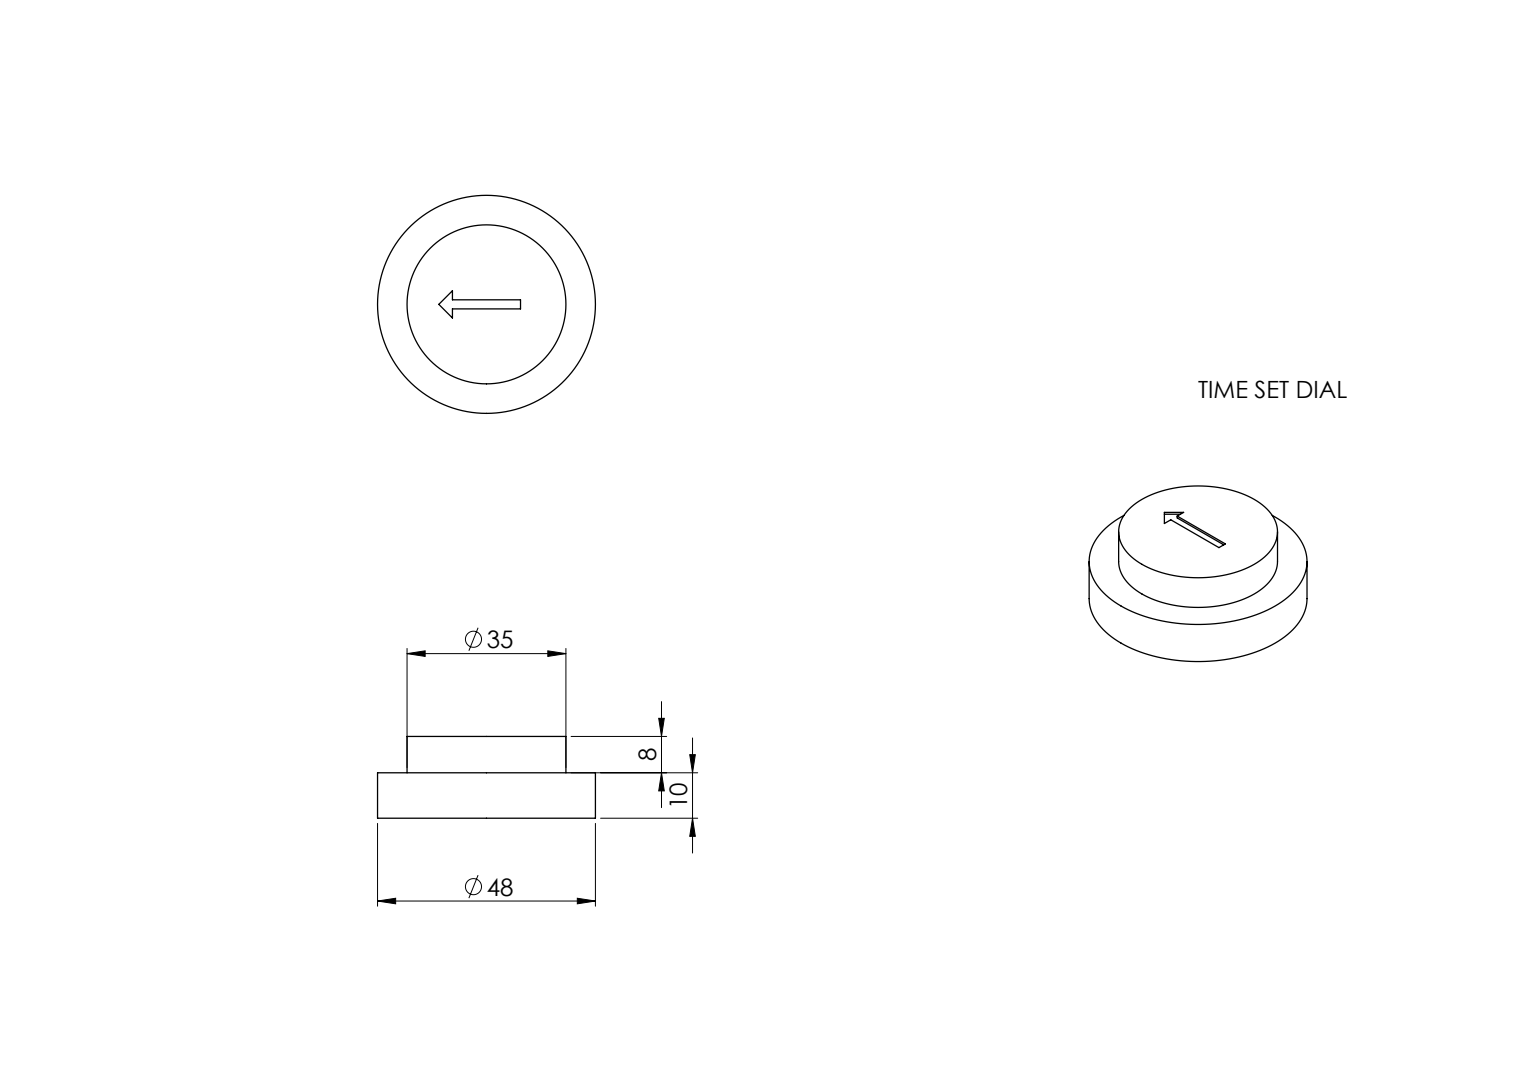
ISO-10303-21;
HEADER;
FILE_DESCRIPTION (('STEP AP214'),
    '1' );
FILE_NAME ('time set dial.step',
    '2026-10-24T15:06:47',
    ( '' ),
    ( '' ),
    'SwSTEP 2.0',
    'SolidWorks 2026',
    '' );
FILE_SCHEMA (( 'AUTOMOTIVE_DESIGN' ));
ENDSEC;

DATA;
#24=FACE_OUTER_BOUND ( 'NONE', #4526, .T. ) ;
#82=AXIS2_PLACEMENT_3D ( 'NONE', #9543, #4773, #8119 ) ;
#92=ORIENTED_EDGE ( 'NONE', *, *, #2350, .T. ) ;
#107=DIRECTION ( 'NONE',  ( 0.000000000000000000, 0.000000000000000000, 1.000000000000000000 ) ) ;
#109=DIRECTION ( 'NONE',  ( 4.336808689942017736E-16, 0.000000000000000000, -1.000000000000000000 ) ) ;
#117=FACE_OUTER_BOUND ( 'NONE', #7334, .T. ) ;
#145=LINE ( 'NONE', #6521, #2502 ) ;
#146=DIRECTION ( 'NONE',  ( -1.000000000000000000, -0.000000000000000000, -0.000000000000000000 ) ) ;
#204=VECTOR ( 'NONE', #9185, 1000.000000000000000 ) ;
#241=ORIENTED_EDGE ( 'NONE', *, *, #4209, .F. ) ;
#262=LINE ( 'NONE', #2027, #6876 ) ;
#291=DIRECTION ( 'NONE',  ( -0.000000000000000000, 1.000000000000000000, -0.000000000000000000 ) ) ;
#295=CIRCLE ( 'NONE', #9511, 17.50000000000000355 ) ;
#305=AXIS2_PLACEMENT_3D ( 'NONE', #9568, #7104, #7052 ) ;
#342=CARTESIAN_POINT ( 'NONE',  ( -10.49999999999999822, 105.0000000000000142, 0.000000000000000000 ) ) ;
#376=CARTESIAN_POINT ( 'NONE',  ( -7.500000000000000000, 105.0000000000000142, 1.000000000000000222 ) ) ;
#379=AXIS2_PLACEMENT_3D ( 'NONE', #1311, #2259, #3050 ) ;
#382=ORIENTED_EDGE ( 'NONE', *, *, #7990, .T. ) ;
#469=LINE ( 'NONE', #7744, #6933 ) ;
#510=STYLED_ITEM('',(#10415),#6220);
#513=PLANE ( 'NONE',  #9858 ) ;
#568=CARTESIAN_POINT ( 'NONE',  ( 7.500000000000000000, 104.5000000000000142, -0.9999999999999997780 ) ) ;
#570=VERTEX_POINT ( 'NONE', #7174 ) ;
#582=PLANE ( 'NONE',  #8912 ) ;
#591=LINE ( 'NONE', #8435, #9453 ) ;
#592=EDGE_CURVE ( 'NONE', #4647, #7571, #9632, .T. ) ;
#595=ORIENTED_EDGE ( 'NONE', *, *, #7990, .F. ) ;
#619=ORIENTED_EDGE ( 'NONE', *, *, #3800, .T. ) ;
#638=ADVANCED_FACE ( 'NONE', ( #8160 ), #1037, .F. ) ;
#674=ORIENTED_EDGE ( 'NONE', *, *, #7210, .F. ) ;
#677=EDGE_LOOP ( 'NONE', ( #674, #3279, #3413, #7812 ) ) ;
#714=ORIENTED_EDGE ( 'NONE', *, *, #1547, .T. ) ;
#726=PLANE ( 'NONE',  #305 ) ;
#741=DIRECTION ( 'NONE',  ( -0.7071067811865476838, 0.000000000000000000, -0.7071067811865474617 ) ) ;
#765=CARTESIAN_POINT ( 'NONE',  ( -7.500000000000000000, 104.5000000000000142, -3.000000000000000000 ) ) ;
#771=VECTOR ( 'NONE', #1661, 1000.000000000000000 ) ;
#781=DIRECTION ( 'NONE',  ( 0.000000000000000000, 1.000000000000000000, 0.000000000000000000 ) ) ;
#794=LINE ( 'NONE', #1520, #8161 ) ;
#808=ORIENTED_EDGE ( 'NONE', *, *, #8492, .T. ) ;
#814=AXIS2_PLACEMENT_3D ( 'NONE', #8760, #6354, #2424 ) ;
#816=DIRECTION ( 'NONE',  ( 0.000000000000000000, 1.000000000000000000, 0.000000000000000000 ) ) ;
#857=ORIENTED_EDGE ( 'NONE', *, *, #9277, .F. ) ;
#864=LINE ( 'NONE', #8915, #7733 ) ;
#906=VERTEX_POINT ( 'NONE', #10349 ) ;
#944=ADVANCED_FACE ( 'NONE', ( #24 ), #4011, .F. ) ;
#960=DIRECTION ( 'NONE',  ( -0.000000000000000000, -1.000000000000000000, -0.000000000000000000 ) ) ;
#1026=PLANE ( 'NONE',  #6043 ) ;
#1036=AXIS2_PLACEMENT_3D ( 'NONE', #6464, #816, #8134 ) ;
#1037=PLANE ( 'NONE',  #7108 ) ;
#1061=VERTEX_POINT ( 'NONE', #376 ) ;
#1093=AXIS2_PLACEMENT_3D ( 'NONE', #5684, #7295, #9604 ) ;
#1097=DIRECTION ( 'NONE',  ( -0.000000000000000000, -1.000000000000000000, -0.000000000000000000 ) ) ;
#1119=LINE ( 'NONE', #1995, #2870 ) ;
#1179=DIRECTION ( 'NONE',  ( 0.7071067811865473507, 0.000000000000000000, 0.7071067811865477948 ) ) ;
#1211=SHAPE_REPRESENTATION_RELATIONSHIP ( 'NONE' , 'NONE' ,  #5481, #6379 ) ;
#1262=CARTESIAN_POINT ( 'NONE',  ( 0.000000000000000000, 97.00000000000000000, 0.000000000000000000 ) ) ;
#1292=CARTESIAN_POINT ( 'NONE',  ( 0.000000000000000000, 105.0000000000000142, 0.000000000000000000 ) ) ;
#1297=ORIENTED_EDGE ( 'NONE', *, *, #1332, .F. ) ;
#1308=UNCERTAINTY_MEASURE_WITH_UNIT (LENGTH_MEASURE( 1.000000000000000082E-05 ), #6022, 'distance_accuracy_value', 'NONE');
#1311=CARTESIAN_POINT ( 'NONE',  ( 0.000000000000000000, 105.0000000000000142, 0.000000000000000000 ) ) ;
#1332=EDGE_CURVE ( 'NONE', #9169, #7011, #4267, .T. ) ;
#1333=PRODUCT ( 'time set dial', 'time set dial', '', ( #2137 ) ) ;
#1352=EDGE_CURVE ( 'NONE', #1061, #570, #8955, .T. ) ;
#1361=CARTESIAN_POINT ( 'NONE',  ( 2.939152317953648289E-15, 97.00000000000000000, 24.00000000000000355 ) ) ;
#1376=ORIENTED_EDGE ( 'NONE', *, *, #1332, .T. ) ;
#1396=( GEOMETRIC_REPRESENTATION_CONTEXT ( 3 ) GLOBAL_UNCERTAINTY_ASSIGNED_CONTEXT ( ( #3296 ) ) GLOBAL_UNIT_ASSIGNED_CONTEXT ( ( #7429, #6752, #9893 ) ) REPRESENTATION_CONTEXT ( 'NONE', 'WORKASPACE' ) );
#1397=PLANE ( 'NONE',  #7889 ) ;
#1403=FACE_OUTER_BOUND ( 'NONE', #9984, .T. ) ;
#1500=CARTESIAN_POINT ( 'NONE',  ( 0.000000000000000000, 105.0000000000000142, -17.50000000000000355 ) ) ;
#1520=CARTESIAN_POINT ( 'NONE',  ( 7.500000000000000000, 104.5000000000000142, 1.000000000000000222 ) ) ;
#1536=ORIENTED_EDGE ( 'NONE', *, *, #7153, .T. ) ;
#1545=ORIENTED_EDGE ( 'NONE', *, *, #9344, .F. ) ;
#1547=EDGE_CURVE ( 'NONE', #7571, #1061, #262, .T. ) ;
#1622=ORIENTED_EDGE ( 'NONE', *, *, #7157, .F. ) ;
#1661=DIRECTION ( 'NONE',  ( -0.000000000000000000, 1.000000000000000000, -0.000000000000000000 ) ) ;
#1675=DIRECTION ( 'NONE',  ( 0.000000000000000000, 0.000000000000000000, -1.000000000000000000 ) ) ;
#1681=DIRECTION ( 'NONE',  ( 0.000000000000000000, 1.000000000000000000, 0.000000000000000000 ) ) ;
#1704=AXIS2_PLACEMENT_3D ( 'NONE', #8807, #9734, #5767 ) ;
#1709=DIRECTION ( 'NONE',  ( 0.000000000000000000, -0.000000000000000000, 1.000000000000000000 ) ) ;
#1720=AXIS2_PLACEMENT_3D ( 'NONE', #9929, #1813, #4230 ) ;
#1727=ORIENTED_EDGE ( 'NONE', *, *, #7157, .T. ) ;
#1743=ORIENTED_EDGE ( 'NONE', *, *, #8141, .F. ) ;
#1753=CARTESIAN_POINT ( 'NONE',  ( -7.500000000000000000, 104.5000000000000142, -3.000000000000000000 ) ) ;
#1761=LINE ( 'NONE', #9094, #8320 ) ;
#1767=CIRCLE ( 'NONE', #1936, 24.00000000000000355 ) ;
#1772=CARTESIAN_POINT ( 'NONE',  ( -7.500000000000000000, 105.0000000000000142, 1.000000000000000222 ) ) ;
#1813=DIRECTION ( 'NONE',  ( 0.000000000000000000, -1.000000000000000000, 0.000000000000000000 ) ) ;
#1837=ORIENTED_EDGE ( 'NONE', *, *, #10080, .F. ) ;
#1865=ORIENTED_EDGE ( 'NONE', *, *, #1352, .T. ) ;
#1898=LINE ( 'NONE', #1753, #5297 ) ;
#1904=DIRECTION ( 'NONE',  ( -0.7071067811865477948, 0.000000000000000000, 0.7071067811865473507 ) ) ;
#1936=AXIS2_PLACEMENT_3D ( 'NONE', #4316, #1681, #9133 ) ;
#1963=( NAMED_UNIT ( * ) PLANE_ANGLE_UNIT ( ) SI_UNIT ( $, .RADIAN. ) );
#1995=CARTESIAN_POINT ( 'NONE',  ( -7.500000000000000000, 104.5000000000000142, -0.9999999999999997780 ) ) ;
#2021=EDGE_CURVE ( 'NONE', #3170, #3531, #7292, .T. ) ;
#2027=CARTESIAN_POINT ( 'NONE',  ( -7.500000000000000000, 104.5000000000000142, 1.000000000000000222 ) ) ;
#2042=PRESENTATION_STYLE_ASSIGNMENT (( #5414 ) ) ;
#2090=AXIS2_PLACEMENT_3D ( 'NONE', #7524, #1097, #5813 ) ;
#2117=AXIS2_PLACEMENT_3D ( 'NONE', #2132, #2192, #6052 ) ;
#2131=VERTEX_POINT ( 'NONE', #2333 ) ;
#2132=CARTESIAN_POINT ( 'NONE',  ( 0.000000000000000000, 87.00000000000001421, 0.000000000000000000 ) ) ;
#2137=PRODUCT_CONTEXT ( 'NONE', #5679, 'mechanical' ) ;
#2149=CARTESIAN_POINT ( 'NONE',  ( -10.49999999999999822, 104.5000000000000142, 0.000000000000000000 ) ) ;
#2158=EDGE_CURVE ( 'NONE', #3256, #2131, #3898, .T. ) ;
#2192=DIRECTION ( 'NONE',  ( 0.000000000000000000, 1.000000000000000000, 0.000000000000000000 ) ) ;
#2259=DIRECTION ( 'NONE',  ( 0.000000000000000000, 1.000000000000000000, 0.000000000000000000 ) ) ;
#2275=ORIENTED_EDGE ( 'NONE', *, *, #6709, .F. ) ;
#2290=CARTESIAN_POINT ( 'NONE',  ( -10.49999999999999822, 104.5000000000000142, 0.000000000000000000 ) ) ;
#2333=CARTESIAN_POINT ( 'NONE',  ( 2.143131898507868643E-15, 97.00000000000000000, 17.50000000000000355 ) ) ;
#2350=EDGE_CURVE ( 'NONE', #6922, #2378, #7401, .T. ) ;
#2360=ADVANCED_FACE ( 'NONE', ( #9865 ), #1026, .F. ) ;
#2378=VERTEX_POINT ( 'NONE', #7452 ) ;
#2393=DIRECTION ( 'NONE',  ( 0.7071067811865473507, 0.000000000000000000, 0.7071067811865477948 ) ) ;
#2394=CARTESIAN_POINT ( 'NONE',  ( 0.000000000000000000, 105.0000000000000142, -17.50000000000000355 ) ) ;
#2424=DIRECTION ( 'NONE',  ( 0.000000000000000000, 0.000000000000000000, -1.000000000000000000 ) ) ;
#2438=EDGE_LOOP ( 'NONE', ( #1622, #7880, #10051, #8233 ) ) ;
#2440=ORIENTED_EDGE ( 'NONE', *, *, #10080, .T. ) ;
#2451=( NAMED_UNIT ( * ) SI_UNIT ( $, .STERADIAN. ) SOLID_ANGLE_UNIT ( ) );
#2464=CARTESIAN_POINT ( 'NONE',  ( -10.49999999999999822, 105.0000000000000142, 0.000000000000000000 ) ) ;
#2466=CARTESIAN_POINT ( 'NONE',  ( -7.500000000000000888, 104.5000000000000142, 3.000000000000000000 ) ) ;
#2501=DIRECTION ( 'NONE',  ( -0.000000000000000000, -0.000000000000000000, -1.000000000000000000 ) ) ;
#2502=VECTOR ( 'NONE', #2501, 1000.000000000000000 ) ;
#2516=CARTESIAN_POINT ( 'NONE',  ( 7.500000000000000000, 104.5000000000000142, 1.000000000000000222 ) ) ;
#2693=EDGE_LOOP ( 'NONE', ( #5365, #6331, #9868, #9244 ) ) ;
#2699=ORIENTED_EDGE ( 'NONE', *, *, #7028, .T. ) ;
#2728=COLOUR_RGB ( '',0.8941176470588234615, 0.8941176470588234615, 0.8941176470588234615 ) ;
#2808=CARTESIAN_POINT ( 'NONE',  ( -10.49999999999999822, 104.5000000000000142, 0.000000000000000000 ) ) ;
#2851=ADVANCED_FACE ( 'NONE', ( #10321, #3724 ), #3106, .T. ) ;
#2861=ADVANCED_FACE ( 'NONE', ( #3775 ), #582, .F. ) ;
#2870=VECTOR ( 'NONE', #5879, 1000.000000000000000 ) ;
#2932=CARTESIAN_POINT ( 'NONE',  ( -7.500000000000000888, 104.5000000000000142, 3.000000000000000000 ) ) ;
#2959=ORIENTED_EDGE ( 'NONE', *, *, #2158, .F. ) ;
#2981=CARTESIAN_POINT ( 'NONE',  ( -7.500000000000000000, 104.5000000000000142, -0.9999999999999997780 ) ) ;
#2999=VECTOR ( 'NONE', #146, 1000.000000000000000 ) ;
#3009=SURFACE_SIDE_STYLE ('',( #5181 ) ) ;
#3050=DIRECTION ( 'NONE',  ( 0.000000000000000000, -0.000000000000000000, 1.000000000000000000 ) ) ;
#3055=ADVANCED_FACE ( 'NONE', ( #9193 ), #8257, .F. ) ;
#3086=ORIENTED_EDGE ( 'NONE', *, *, #3800, .F. ) ;
#3103=PRODUCT_DEFINITION_CONTEXT ( 'detailed design', #10152, 'design' ) ;
#3106=PLANE ( 'NONE',  #379 ) ;
#3143=DIRECTION ( 'NONE',  ( 0.000000000000000000, 0.000000000000000000, 1.000000000000000000 ) ) ;
#3170=VERTEX_POINT ( 'NONE', #10067 ) ;
#3183=DIRECTION ( 'NONE',  ( -0.000000000000000000, -1.000000000000000000, -0.000000000000000000 ) ) ;
#3256=VERTEX_POINT ( 'NONE', #8560 ) ;
#3279=ORIENTED_EDGE ( 'NONE', *, *, #6211, .F. ) ;
#3296=UNCERTAINTY_MEASURE_WITH_UNIT (LENGTH_MEASURE( 1.000000000000000082E-05 ), #7429, 'distance_accuracy_value', 'NONE');
#3327=DIRECTION ( 'NONE',  ( 0.000000000000000000, 0.000000000000000000, 1.000000000000000000 ) ) ;
#3329=EDGE_CURVE ( 'NONE', #9169, #9715, #864, .T. ) ;
#3398=CYLINDRICAL_SURFACE ( 'NONE', #2090, 17.50000000000000355 ) ;
#3401=ORIENTED_EDGE ( 'NONE', *, *, #592, .T. ) ;
#3413=ORIENTED_EDGE ( 'NONE', *, *, #9332, .T. ) ;
#3442=PRODUCT_DEFINITION ( 'UNKNOWN', '', #8308, #3103 ) ;
#3453=AXIS2_PLACEMENT_3D ( 'NONE', #4025, #781, #3143 ) ;
#3457=EDGE_LOOP ( 'NONE', ( #9362, #5000, #7737, #2440 ) ) ;
#3495=VERTEX_POINT ( 'NONE', #7941 ) ;
#3527=CARTESIAN_POINT ( 'NONE',  ( -10.49999999999999822, 105.0000000000000142, 0.000000000000000000 ) ) ;
#3531=VERTEX_POINT ( 'NONE', #10354 ) ;
#3541=LINE ( 'NONE', #2516, #9546 ) ;
#3580=ADVANCED_FACE ( 'NONE', ( #5380 ), #1397, .F. ) ;
#3611=DIRECTION ( 'NONE',  ( -0.000000000000000000, 1.000000000000000000, -0.000000000000000000 ) ) ;
#3618=AXIS2_PLACEMENT_3D ( 'NONE', #3964, #9514, #3327 ) ;
#3648=CIRCLE ( 'NONE', #7997, 17.50000000000000355 ) ;
#3653=DIRECTION ( 'NONE',  ( 0.000000000000000000, 0.000000000000000000, -1.000000000000000000 ) ) ;
#3680=EDGE_LOOP ( 'NONE', ( #9796, #7586, #241, #5335, #3732, #5188, #9994 ) ) ;
#3724=FACE_OUTER_BOUND ( 'NONE', #9122, .T. ) ;
#3732=ORIENTED_EDGE ( 'NONE', *, *, #7105, .F. ) ;
#3762=PLANE ( 'NONE',  #2117 ) ;
#3775=FACE_OUTER_BOUND ( 'NONE', #9335, .T. ) ;
#3781=ORIENTED_EDGE ( 'NONE', *, *, #8141, .T. ) ;
#3790=ORIENTED_EDGE ( 'NONE', *, *, #8261, .F. ) ;
#3800=EDGE_CURVE ( 'NONE', #7095, #2378, #1119, .T. ) ;
#3801=CIRCLE ( 'NONE', #3618, 24.00000000000000355 ) ;
#3813=ORIENTED_EDGE ( 'NONE', *, *, #2021, .T. ) ;
#3822=VECTOR ( 'NONE', #8896, 1000.000000000000000 ) ;
#3893=ORIENTED_EDGE ( 'NONE', *, *, #7153, .F. ) ;
#3898=CIRCLE ( 'NONE', #1036, 17.50000000000000355 ) ;
#3934=DIRECTION ( 'NONE',  ( -0.7071067811865474617, 0.000000000000000000, 0.7071067811865476838 ) ) ;
#3964=CARTESIAN_POINT ( 'NONE',  ( 0.000000000000000000, 87.00000000000001421, 0.000000000000000000 ) ) ;
#3985=DIRECTION ( 'NONE',  ( 0.000000000000000000, 1.000000000000000000, 0.000000000000000000 ) ) ;
#4011=PLANE ( 'NONE',  #1093 ) ;
#4025=CARTESIAN_POINT ( 'NONE',  ( 0.000000000000000000, 87.00000000000001421, 0.000000000000000000 ) ) ;
#4055=VECTOR ( 'NONE', #4095, 1000.000000000000000 ) ;
#4068=MECHANICAL_DESIGN_GEOMETRIC_PRESENTATION_REPRESENTATION('',(#7237),#7083);
#4095=DIRECTION ( 'NONE',  ( 1.000000000000000000, 0.000000000000000000, 0.000000000000000000 ) ) ;
#4154=DIRECTION ( 'NONE',  ( 0.000000000000000000, 0.000000000000000000, 1.000000000000000000 ) ) ;
#4169=ORIENTED_EDGE ( 'NONE', *, *, #9725, .T. ) ;
#4192=CARTESIAN_POINT ( 'NONE',  ( 0.000000000000000000, 97.00000000000000000, 0.000000000000000000 ) ) ;
#4209=EDGE_CURVE ( 'NONE', #4294, #1061, #591, .T. ) ;
#4216=FACE_OUTER_BOUND ( 'NONE', #6879, .T. ) ;
#4230=DIRECTION ( 'NONE',  ( 0.000000000000000000, -0.000000000000000000, -1.000000000000000000 ) ) ;
#4263=ADVANCED_FACE ( 'NONE', ( #117 ), #5669, .T. ) ;
#4267=CIRCLE ( 'NONE', #1704, 24.00000000000000355 ) ;
#4279=DIRECTION ( 'NONE',  ( 1.000000000000000000, 0.000000000000000000, 4.336808689942017736E-16 ) ) ;
#4294=VERTEX_POINT ( 'NONE', #9639 ) ;
#4311=AXIS2_PLACEMENT_3D ( 'NONE', #9712, #7397, #1709 ) ;
#4316=CARTESIAN_POINT ( 'NONE',  ( 0.000000000000000000, 97.00000000000000000, 0.000000000000000000 ) ) ;
#4420=CARTESIAN_POINT ( 'NONE',  ( -10.49999999999999822, 104.5000000000000142, 0.000000000000000000 ) ) ;
#4451=FACE_OUTER_BOUND ( 'NONE', #8412, .T. ) ;
#4470=CARTESIAN_POINT ( 'NONE',  ( 7.500000000000000000, 104.5000000000000142, -0.9999999999999997780 ) ) ;
#4472=CARTESIAN_POINT ( 'NONE',  ( 0.000000000000000000, 97.00000000000000000, -24.00000000000000355 ) ) ;
#4526=EDGE_LOOP ( 'NONE', ( #5095, #6153, #3790, #619 ) ) ;
#4563=( NAMED_UNIT ( * ) PLANE_ANGLE_UNIT ( ) SI_UNIT ( $, .RADIAN. ) );
#4572=VECTOR ( 'NONE', #291, 1000.000000000000000 ) ;
#4647=VERTEX_POINT ( 'NONE', #2932 ) ;
#4773=DIRECTION ( 'NONE',  ( -0.000000000000000000, -1.000000000000000000, -0.000000000000000000 ) ) ;
#4796=ORIENTED_EDGE ( 'NONE', *, *, #6012, .F. ) ;
#4797=VECTOR ( 'NONE', #109, 1000.000000000000000 ) ;
#4903=VECTOR ( 'NONE', #1179, 999.9999999999998863 ) ;
#4930=DIRECTION ( 'NONE',  ( 0.000000000000000000, 0.000000000000000000, -1.000000000000000000 ) ) ;
#4934=FILL_AREA_STYLE_COLOUR ( '', #2728 ) ;
#4961=CARTESIAN_POINT ( 'NONE',  ( -7.500000000000000888, 104.5000000000000142, 3.000000000000000000 ) ) ;
#5000=ORIENTED_EDGE ( 'NONE', *, *, #5457, .F. ) ;
#5055=AXIS2_PLACEMENT_3D ( 'NONE', #9842, #4154, #9744 ) ;
#5095=ORIENTED_EDGE ( 'NONE', *, *, #6474, .T. ) ;
#5107=EDGE_CURVE ( 'NONE', #7571, #3495, #469, .T. ) ;
#5127=LINE ( 'NONE', #6551, #7444 ) ;
#5181=SURFACE_STYLE_FILL_AREA ( #8132 ) ;
#5188=ORIENTED_EDGE ( 'NONE', *, *, #6474, .F. ) ;
#5200=EDGE_LOOP ( 'NONE', ( #1536, #9622, #9646, #7764, #808, #3401, #7707 ) ) ;
#5297=VECTOR ( 'NONE', #9030, 1000.000000000000000 ) ;
#5299=EDGE_LOOP ( 'NONE', ( #4169, #595, #3893, #9829 ) ) ;
#5330=DIRECTION ( 'NONE',  ( -1.000000000000000000, 0.000000000000000000, -0.000000000000000000 ) ) ;
#5335=ORIENTED_EDGE ( 'NONE', *, *, #10165, .F. ) ;
#5365=ORIENTED_EDGE ( 'NONE', *, *, #4209, .T. ) ;
#5380=FACE_OUTER_BOUND ( 'NONE', #5299, .T. ) ;
#5414=SURFACE_STYLE_USAGE ( .BOTH. , #3009 ) ;
#5457=EDGE_CURVE ( 'NONE', #4647, #4294, #6160, .T. ) ;
#5481=SHAPE_REPRESENTATION ( 'time set dial', ( #5055 ), #1396 ) ;
#5487=LINE ( 'NONE', #8879, #8970 ) ;
#5537=CIRCLE ( 'NONE', #8039, 17.50000000000000355 ) ;
#5621=FACE_OUTER_BOUND ( 'NONE', #2438, .T. ) ;
#5635=AXIS2_PLACEMENT_3D ( 'NONE', #1262, #9889, #7638 ) ;
#5669=CYLINDRICAL_SURFACE ( 'NONE', #82, 24.00000000000000355 ) ;
#5679=APPLICATION_CONTEXT ( 'automotive_design' ) ;
#5684=CARTESIAN_POINT ( 'NONE',  ( -7.500000000000000000, 104.5000000000000142, -3.000000000000000000 ) ) ;
#5711=ADVANCED_FACE ( 'NONE', ( #7474 ), #3398, .T. ) ;
#5767=DIRECTION ( 'NONE',  ( 0.000000000000000000, 0.000000000000000000, 1.000000000000000000 ) ) ;
#5792=VECTOR ( 'NONE', #2393, 999.9999999999998863 ) ;
#5799=DIRECTION ( 'NONE',  ( -0.000000000000000000, 1.000000000000000000, -0.000000000000000000 ) ) ;
#5813=DIRECTION ( 'NONE',  ( 0.000000000000000000, 0.000000000000000000, -1.000000000000000000 ) ) ;
#5835=CARTESIAN_POINT ( 'NONE',  ( -7.500000000000000000, 104.5000000000000142, -0.9999999999999997780 ) ) ;
#5879=DIRECTION ( 'NONE',  ( -0.000000000000000000, 1.000000000000000000, -0.000000000000000000 ) ) ;
#6011=ORIENTED_EDGE ( 'NONE', *, *, #3329, .F. ) ;
#6012=EDGE_CURVE ( 'NONE', #3495, #570, #3541, .T. ) ;
#6022=( LENGTH_UNIT ( ) NAMED_UNIT ( * ) SI_UNIT ( .MILLI., .METRE. ) );
#6043=AXIS2_PLACEMENT_3D ( 'NONE', #2808, #1904, #7558 ) ;
#6052=DIRECTION ( 'NONE',  ( 0.000000000000000000, -0.000000000000000000, 1.000000000000000000 ) ) ;
#6153=ORIENTED_EDGE ( 'NONE', *, *, #2021, .F. ) ;
#6160=LINE ( 'NONE', #9358, #771 ) ;
#6165=FACE_OUTER_BOUND ( 'NONE', #8609, .T. ) ;
#6208=ADVANCED_FACE ( 'NONE', ( #1403 ), #513, .F. ) ;
#6209=DIRECTION ( 'NONE',  ( 0.000000000000000000, 0.000000000000000000, -1.000000000000000000 ) ) ;
#6211=EDGE_CURVE ( 'NONE', #9263, #906, #5537, .T. ) ;
#6220=MANIFOLD_SOLID_BREP ( 'Cut-Extrude1', #6475 ) ;
#6331=ORIENTED_EDGE ( 'NONE', *, *, #1547, .F. ) ;
#6354=DIRECTION ( 'NONE',  ( -0.000000000000000000, -1.000000000000000000, -0.000000000000000000 ) ) ;
#6379=ADVANCED_BREP_SHAPE_REPRESENTATION ( '', ( #6220, #5055 ), #1396 ) ;
#6427=FACE_OUTER_BOUND ( 'NONE', #8772, .T. ) ;
#6464=CARTESIAN_POINT ( 'NONE',  ( 0.000000000000000000, 97.00000000000000000, 0.000000000000000000 ) ) ;
#6474=EDGE_CURVE ( 'NONE', #2378, #3531, #145, .T. ) ;
#6475=CLOSED_SHELL ( 'NONE', ( #6591, #4263, #8882, #7640, #8015, #5711, #2851, #3580, #7442, #638, #2360, #2861, #944, #6208, #3055 ) ) ;
#6494=VERTEX_POINT ( 'NONE', #3527 ) ;
#6521=CARTESIAN_POINT ( 'NONE',  ( -7.500000000000000000, 105.0000000000000142, -3.000000000000000000 ) ) ;
#6549=EDGE_LOOP ( 'NONE', ( #2959, #2275 ) ) ;
#6551=CARTESIAN_POINT ( 'NONE',  ( 7.500000000000000000, 105.0000000000000142, 1.000000000000000222 ) ) ;
#6591=ADVANCED_FACE ( 'NONE', ( #5621 ), #7283, .T. ) ;
#6672=ORIENTED_EDGE ( 'NONE', *, *, #9277, .T. ) ;
#6693=CYLINDRICAL_SURFACE ( 'NONE', #5635, 24.00000000000000355 ) ;
#6709=EDGE_CURVE ( 'NONE', #2131, #3256, #295, .T. ) ;
#6752=( NAMED_UNIT ( * ) PLANE_ANGLE_UNIT ( ) SI_UNIT ( $, .RADIAN. ) );
#6824=CARTESIAN_POINT ( 'NONE',  ( -10.49999999999999822, 104.5000000000000142, 0.000000000000000000 ) ) ;
#6833=DIRECTION ( 'NONE',  ( 0.000000000000000000, 1.000000000000000000, 0.000000000000000000 ) ) ;
#6876=VECTOR ( 'NONE', #3611, 1000.000000000000000 ) ;
#6879=EDGE_LOOP ( 'NONE', ( #1376, #9472 ) ) ;
#6880=LINE ( 'NONE', #6824, #4572 ) ;
#6922=VERTEX_POINT ( 'NONE', #9997 ) ;
#6933=VECTOR ( 'NONE', #9370, 1000.000000000000000 ) ;
#6974=CIRCLE ( 'NONE', #3453, 24.00000000000000355 ) ;
#7011=VERTEX_POINT ( 'NONE', #1361 ) ;
#7019=ORIENTED_EDGE ( 'NONE', *, *, #7028, .F. ) ;
#7022=( NAMED_UNIT ( * ) SI_UNIT ( $, .STERADIAN. ) SOLID_ANGLE_UNIT ( ) );
#7028=EDGE_CURVE ( 'NONE', #7011, #9319, #8481, .T. ) ;
#7052=DIRECTION ( 'NONE',  ( 1.000000000000000000, 0.000000000000000000, 0.000000000000000000 ) ) ;
#7083=( GEOMETRIC_REPRESENTATION_CONTEXT ( 3 ) GLOBAL_UNCERTAINTY_ASSIGNED_CONTEXT ( ( #1308 ) ) GLOBAL_UNIT_ASSIGNED_CONTEXT ( ( #6022, #4563, #7022 ) ) REPRESENTATION_CONTEXT ( 'NONE', 'WORKASPACE' ) );
#7095=VERTEX_POINT ( 'NONE', #8849 ) ;
#7104=DIRECTION ( 'NONE',  ( -0.000000000000000000, 0.000000000000000000, 1.000000000000000000 ) ) ;
#7105=EDGE_CURVE ( 'NONE', #3531, #6494, #8013, .T. ) ;
#7108=AXIS2_PLACEMENT_3D ( 'NONE', #4961, #4279, #7320 ) ;
#7150=CARTESIAN_POINT ( 'NONE',  ( 2.939152317953648289E-15, 87.00000000000001421, 24.00000000000000355 ) ) ;
#7153=EDGE_CURVE ( 'NONE', #3495, #7824, #794, .T. ) ;
#7157=EDGE_CURVE ( 'NONE', #906, #9263, #3648, .T. ) ;
#7174=CARTESIAN_POINT ( 'NONE',  ( 7.500000000000000000, 105.0000000000000142, 1.000000000000000222 ) ) ;
#7191=PRODUCT_DEFINITION_SHAPE ( 'NONE', 'NONE',  #3442 ) ;
#7210=EDGE_CURVE ( 'NONE', #906, #2131, #1761, .T. ) ;
#7237=STYLED_ITEM ( 'NONE', ( #2042 ), #6379 ) ;
#7242=DIRECTION ( 'NONE',  ( -0.000000000000000000, 1.000000000000000000, -0.000000000000000000 ) ) ;
#7283=CYLINDRICAL_SURFACE ( 'NONE', #814, 17.50000000000000355 ) ;
#7292=LINE ( 'NONE', #765, #8061 ) ;
#7295=DIRECTION ( 'NONE',  ( 1.000000000000000000, 0.000000000000000000, -0.000000000000000000 ) ) ;
#7307=CARTESIAN_POINT ( 'NONE',  ( -7.500000000000000000, 104.5000000000000142, 1.000000000000000222 ) ) ;
#7320=DIRECTION ( 'NONE',  ( 4.336808689942017736E-16, 0.000000000000000000, -1.000000000000000000 ) ) ;
#7334=EDGE_LOOP ( 'NONE', ( #10182, #2699, #6672, #6011 ) ) ;
#7397=DIRECTION ( 'NONE',  ( 0.000000000000000000, 1.000000000000000000, 0.000000000000000000 ) ) ;
#7401=LINE ( 'NONE', #9137, #204 ) ;
#7429=( LENGTH_UNIT ( ) NAMED_UNIT ( * ) SI_UNIT ( .MILLI., .METRE. ) );
#7442=ADVANCED_FACE ( 'NONE', ( #6427 ), #726, .F. ) ;
#7444=VECTOR ( 'NONE', #4930, 1000.000000000000000 ) ;
#7445=PLANE ( 'NONE',  #4311 ) ;
#7452=CARTESIAN_POINT ( 'NONE',  ( -7.500000000000000000, 105.0000000000000142, -0.9999999999999997780 ) ) ;
#7474=FACE_OUTER_BOUND ( 'NONE', #677, .T. ) ;
#7524=CARTESIAN_POINT ( 'NONE',  ( 0.000000000000000000, 105.0000000000000142, 0.000000000000000000 ) ) ;
#7558=DIRECTION ( 'NONE',  ( 0.7071067811865473507, 0.000000000000000000, 0.7071067811865477948 ) ) ;
#7571=VERTEX_POINT ( 'NONE', #7307 ) ;
#7586=ORIENTED_EDGE ( 'NONE', *, *, #1352, .F. ) ;
#7638=DIRECTION ( 'NONE',  ( 0.000000000000000000, 0.000000000000000000, -1.000000000000000000 ) ) ;
#7640=ADVANCED_FACE ( 'NONE', ( #8194, #4216 ), #7445, .T. ) ;
#7643=EDGE_CURVE ( 'NONE', #7824, #7095, #8099, .T. ) ;
#7683=SHAPE_DEFINITION_REPRESENTATION ( #7191, #5481 ) ;
#7692=CARTESIAN_POINT ( 'NONE',  ( 2.939152317953648289E-15, 97.00000000000000000, 24.00000000000000355 ) ) ;
#7707=ORIENTED_EDGE ( 'NONE', *, *, #5107, .T. ) ;
#7733=VECTOR ( 'NONE', #960, 1000.000000000000000 ) ;
#7737=ORIENTED_EDGE ( 'NONE', *, *, #8492, .F. ) ;
#7744=CARTESIAN_POINT ( 'NONE',  ( -7.500000000000000000, 104.5000000000000142, 1.000000000000000222 ) ) ;
#7764=ORIENTED_EDGE ( 'NONE', *, *, #9344, .T. ) ;
#7765=VERTEX_POINT ( 'NONE', #4420 ) ;
#7779=DIRECTION ( 'NONE',  ( 1.000000000000000000, 0.000000000000000000, 0.000000000000000000 ) ) ;
#7812=ORIENTED_EDGE ( 'NONE', *, *, #2158, .T. ) ;
#7824=VERTEX_POINT ( 'NONE', #4470 ) ;
#7845=LINE ( 'NONE', #568, #8471 ) ;
#7880=ORIENTED_EDGE ( 'NONE', *, *, #7210, .T. ) ;
#7885=ORIENTED_EDGE ( 'NONE', *, *, #6211, .T. ) ;
#7889=AXIS2_PLACEMENT_3D ( 'NONE', #9515, #7779, #6209 ) ;
#7941=CARTESIAN_POINT ( 'NONE',  ( 7.500000000000000000, 104.5000000000000142, 1.000000000000000222 ) ) ;
#7990=EDGE_CURVE ( 'NONE', #7824, #6922, #7845, .T. ) ;
#7997=AXIS2_PLACEMENT_3D ( 'NONE', #8797, #3985, #107 ) ;
#8013=LINE ( 'NONE', #2464, #3822 ) ;
#8015=ADVANCED_FACE ( 'NONE', ( #6165 ), #3762, .F. ) ;
#8039=AXIS2_PLACEMENT_3D ( 'NONE', #1292, #6833, #8520 ) ;
#8061=VECTOR ( 'NONE', #7242, 1000.000000000000000 ) ;
#8099=LINE ( 'NONE', #5835, #2999 ) ;
#8119=DIRECTION ( 'NONE',  ( 0.000000000000000000, 0.000000000000000000, -1.000000000000000000 ) ) ;
#8132=FILL_AREA_STYLE ('',( #4934 ) ) ;
#8134=DIRECTION ( 'NONE',  ( 0.000000000000000000, 0.000000000000000000, 1.000000000000000000 ) ) ;
#8141=EDGE_CURVE ( 'NONE', #9715, #9319, #6974, .T. ) ;
#8160=FACE_OUTER_BOUND ( 'NONE', #2693, .T. ) ;
#8161=VECTOR ( 'NONE', #1675, 1000.000000000000000 ) ;
#8175=CARTESIAN_POINT ( 'NONE',  ( 0.000000000000000000, 87.00000000000001421, -24.00000000000000355 ) ) ;
#8194=FACE_BOUND ( 'NONE', #6549, .T. ) ;
#8233=ORIENTED_EDGE ( 'NONE', *, *, #9332, .F. ) ;
#8257=PLANE ( 'NONE',  #1720 ) ;
#8261=EDGE_CURVE ( 'NONE', #7095, #3170, #1898, .T. ) ;
#8308=PRODUCT_DEFINITION_FORMATION_WITH_SPECIFIED_SOURCE ( 'ANY', '', #1333, .NOT_KNOWN. ) ;
#8320=VECTOR ( 'NONE', #9928, 1000.000000000000000 ) ;
#8363=MECHANICAL_DESIGN_GEOMETRIC_PRESENTATION_REPRESENTATION('',(#510),#8877);
#8412=EDGE_LOOP ( 'NONE', ( #7019, #1297, #10007, #3781 ) ) ;
#8435=CARTESIAN_POINT ( 'NONE',  ( -7.500000000000000888, 105.0000000000000142, 3.000000000000000000 ) ) ;
#8471=VECTOR ( 'NONE', #10149, 1000.000000000000000 ) ;
#8481=LINE ( 'NONE', #7692, #9666 ) ;
#8492=EDGE_CURVE ( 'NONE', #7765, #4647, #8729, .T. ) ;
#8520=DIRECTION ( 'NONE',  ( 0.000000000000000000, 0.000000000000000000, 1.000000000000000000 ) ) ;
#8547=DIRECTION ( 'NONE',  ( 4.336808689942017736E-16, 0.000000000000000000, -1.000000000000000000 ) ) ;
#8560=CARTESIAN_POINT ( 'NONE',  ( 0.000000000000000000, 97.00000000000000000, -17.50000000000000355 ) ) ;
#8596=DIRECTION ( 'NONE',  ( -0.000000000000000000, -1.000000000000000000, -0.000000000000000000 ) ) ;
#8609=EDGE_LOOP ( 'NONE', ( #1743, #857 ) ) ;
#8729=LINE ( 'NONE', #2290, #5792 ) ;
#8760=CARTESIAN_POINT ( 'NONE',  ( 0.000000000000000000, 105.0000000000000142, 0.000000000000000000 ) ) ;
#8762=ORIENTED_EDGE ( 'NONE', *, *, #7643, .F. ) ;
#8772=EDGE_LOOP ( 'NONE', ( #1865, #4796, #8780, #714 ) ) ;
#8780=ORIENTED_EDGE ( 'NONE', *, *, #5107, .F. ) ;
#8797=CARTESIAN_POINT ( 'NONE',  ( 0.000000000000000000, 105.0000000000000142, 0.000000000000000000 ) ) ;
#8807=CARTESIAN_POINT ( 'NONE',  ( 0.000000000000000000, 97.00000000000000000, 0.000000000000000000 ) ) ;
#8849=CARTESIAN_POINT ( 'NONE',  ( -7.500000000000000000, 104.5000000000000142, -0.9999999999999997780 ) ) ;
#8877=( GEOMETRIC_REPRESENTATION_CONTEXT ( 3 ) GLOBAL_UNCERTAINTY_ASSIGNED_CONTEXT ( ( #9483 ) ) GLOBAL_UNIT_ASSIGNED_CONTEXT ( ( #10146, #1963, #2451 ) ) REPRESENTATION_CONTEXT ( 'NONE', 'WORKASPACE' ) );
#8879=CARTESIAN_POINT ( 'NONE',  ( -10.49999999999999822, 104.5000000000000142, 0.000000000000000000 ) ) ;
#8882=ADVANCED_FACE ( 'NONE', ( #4451 ), #6693, .T. ) ;
#8896=DIRECTION ( 'NONE',  ( -0.7071067811865474617, -0.000000000000000000, 0.7071067811865476838 ) ) ;
#8912=AXIS2_PLACEMENT_3D ( 'NONE', #2149, #741, #3934 ) ;
#8915=CARTESIAN_POINT ( 'NONE',  ( 0.000000000000000000, 97.00000000000000000, -24.00000000000000355 ) ) ;
#8955=LINE ( 'NONE', #1772, #4055 ) ;
#8970=VECTOR ( 'NONE', #9563, 1000.000000000000000 ) ;
#9027=EDGE_CURVE ( 'NONE', #7011, #9169, #1767, .T. ) ;
#9030=DIRECTION ( 'NONE',  ( -0.000000000000000000, -0.000000000000000000, -1.000000000000000000 ) ) ;
#9057=DIRECTION ( 'NONE',  ( 0.000000000000000000, 0.000000000000000000, 1.000000000000000000 ) ) ;
#9094=CARTESIAN_POINT ( 'NONE',  ( 2.143131898507868643E-15, 105.0000000000000142, 17.50000000000000355 ) ) ;
#9122=EDGE_LOOP ( 'NONE', ( #7885, #1727 ) ) ;
#9133=DIRECTION ( 'NONE',  ( 0.000000000000000000, 0.000000000000000000, 1.000000000000000000 ) ) ;
#9137=CARTESIAN_POINT ( 'NONE',  ( -7.500000000000000000, 105.0000000000000142, -0.9999999999999997780 ) ) ;
#9169=VERTEX_POINT ( 'NONE', #4472 ) ;
#9185=DIRECTION ( 'NONE',  ( -1.000000000000000000, -0.000000000000000000, -0.000000000000000000 ) ) ;
#9193=FACE_OUTER_BOUND ( 'NONE', #5200, .T. ) ;
#9244=ORIENTED_EDGE ( 'NONE', *, *, #5457, .T. ) ;
#9263=VERTEX_POINT ( 'NONE', #1500 ) ;
#9277=EDGE_CURVE ( 'NONE', #9319, #9715, #3801, .T. ) ;
#9319=VERTEX_POINT ( 'NONE', #7150 ) ;
#9332=EDGE_CURVE ( 'NONE', #9263, #3256, #10353, .T. ) ;
#9335=EDGE_LOOP ( 'NONE', ( #9614, #1837, #1545, #3813 ) ) ;
#9344=EDGE_CURVE ( 'NONE', #3170, #7765, #5487, .T. ) ;
#9358=CARTESIAN_POINT ( 'NONE',  ( -7.500000000000000888, 104.5000000000000142, 3.000000000000000000 ) ) ;
#9362=ORIENTED_EDGE ( 'NONE', *, *, #10165, .T. ) ;
#9370=DIRECTION ( 'NONE',  ( 1.000000000000000000, 0.000000000000000000, 0.000000000000000000 ) ) ;
#9453=VECTOR ( 'NONE', #8547, 1000.000000000000000 ) ;
#9472=ORIENTED_EDGE ( 'NONE', *, *, #9027, .T. ) ;
#9483=UNCERTAINTY_MEASURE_WITH_UNIT (LENGTH_MEASURE( 1.000000000000000082E-05 ), #10146, 'distance_accuracy_value', 'NONE');
#9511=AXIS2_PLACEMENT_3D ( 'NONE', #4192, #9943, #9057 ) ;
#9514=DIRECTION ( 'NONE',  ( 0.000000000000000000, 1.000000000000000000, 0.000000000000000000 ) ) ;
#9515=CARTESIAN_POINT ( 'NONE',  ( 7.500000000000000000, 104.5000000000000142, 1.000000000000000222 ) ) ;
#9543=CARTESIAN_POINT ( 'NONE',  ( 0.000000000000000000, 97.00000000000000000, 0.000000000000000000 ) ) ;
#9546=VECTOR ( 'NONE', #5799, 1000.000000000000000 ) ;
#9563=DIRECTION ( 'NONE',  ( -0.7071067811865474617, -0.000000000000000000, 0.7071067811865476838 ) ) ;
#9568=CARTESIAN_POINT ( 'NONE',  ( -7.500000000000000000, 104.5000000000000142, 1.000000000000000222 ) ) ;
#9604=DIRECTION ( 'NONE',  ( -0.000000000000000000, 0.000000000000000000, -1.000000000000000000 ) ) ;
#9614=ORIENTED_EDGE ( 'NONE', *, *, #7105, .T. ) ;
#9622=ORIENTED_EDGE ( 'NONE', *, *, #7643, .T. ) ;
#9632=LINE ( 'NONE', #2466, #4797 ) ;
#9639=CARTESIAN_POINT ( 'NONE',  ( -7.500000000000000888, 105.0000000000000142, 3.000000000000000000 ) ) ;
#9646=ORIENTED_EDGE ( 'NONE', *, *, #8261, .T. ) ;
#9666=VECTOR ( 'NONE', #8596, 1000.000000000000000 ) ;
#9712=CARTESIAN_POINT ( 'NONE',  ( 0.000000000000000000, 97.00000000000000000, 0.000000000000000000 ) ) ;
#9715=VERTEX_POINT ( 'NONE', #8175 ) ;
#9725=EDGE_CURVE ( 'NONE', #570, #6922, #5127, .T. ) ;
#9734=DIRECTION ( 'NONE',  ( 0.000000000000000000, 1.000000000000000000, 0.000000000000000000 ) ) ;
#9744=DIRECTION ( 'NONE',  ( 1.000000000000000000, 0.000000000000000000, 0.000000000000000000 ) ) ;
#9796=ORIENTED_EDGE ( 'NONE', *, *, #9725, .F. ) ;
#9829=ORIENTED_EDGE ( 'NONE', *, *, #6012, .T. ) ;
#9842=CARTESIAN_POINT ( 'NONE',  ( 0.000000000000000000, 0.000000000000000000, 0.000000000000000000 ) ) ;
#9858=AXIS2_PLACEMENT_3D ( 'NONE', #2981, #3653, #5330 ) ;
#9863=LINE ( 'NONE', #342, #4903 ) ;
#9865=FACE_OUTER_BOUND ( 'NONE', #3457, .T. ) ;
#9868=ORIENTED_EDGE ( 'NONE', *, *, #592, .F. ) ;
#9889=DIRECTION ( 'NONE',  ( -0.000000000000000000, -1.000000000000000000, -0.000000000000000000 ) ) ;
#9893=( NAMED_UNIT ( * ) SI_UNIT ( $, .STERADIAN. ) SOLID_ANGLE_UNIT ( ) );
#9928=DIRECTION ( 'NONE',  ( -0.000000000000000000, -1.000000000000000000, -0.000000000000000000 ) ) ;
#9929=CARTESIAN_POINT ( 'NONE',  ( 0.000000000000000000, 104.5000000000000142, 0.000000000000000000 ) ) ;
#9943=DIRECTION ( 'NONE',  ( 0.000000000000000000, 1.000000000000000000, 0.000000000000000000 ) ) ;
#9984=EDGE_LOOP ( 'NONE', ( #92, #3086, #8762, #382 ) ) ;
#9994=ORIENTED_EDGE ( 'NONE', *, *, #2350, .F. ) ;
#9997=CARTESIAN_POINT ( 'NONE',  ( 7.500000000000000000, 105.0000000000000142, -0.9999999999999997780 ) ) ;
#10007=ORIENTED_EDGE ( 'NONE', *, *, #3329, .T. ) ;
#10051=ORIENTED_EDGE ( 'NONE', *, *, #6709, .T. ) ;
#10067=CARTESIAN_POINT ( 'NONE',  ( -7.500000000000000000, 104.5000000000000142, -3.000000000000000000 ) ) ;
#10080=EDGE_CURVE ( 'NONE', #7765, #6494, #6880, .T. ) ;
#10146=( LENGTH_UNIT ( ) NAMED_UNIT ( * ) SI_UNIT ( .MILLI., .METRE. ) );
#10149=DIRECTION ( 'NONE',  ( -0.000000000000000000, 1.000000000000000000, -0.000000000000000000 ) ) ;
#10152=APPLICATION_CONTEXT ( 'automotive_design' ) ;
#10165=EDGE_CURVE ( 'NONE', #6494, #4294, #9863, .T. ) ;
#10182=ORIENTED_EDGE ( 'NONE', *, *, #9027, .F. ) ;
#10313=VECTOR ( 'NONE', #3183, 1000.000000000000000 ) ;
#10321=FACE_BOUND ( 'NONE', #3680, .T. ) ;
#10349=CARTESIAN_POINT ( 'NONE',  ( 2.143131898507868643E-15, 105.0000000000000142, 17.50000000000000355 ) ) ;
#10353=LINE ( 'NONE', #2394, #10313 ) ;
#10354=CARTESIAN_POINT ( 'NONE',  ( -7.500000000000000000, 105.0000000000000142, -3.000000000000000000 ) ) ;
#10409=COLOUR_RGB('Off White',0.89,0.88,0.83);
#10410=FILL_AREA_STYLE_COLOUR('',#10409);
#10411=FILL_AREA_STYLE('',(#10410));
#10412=SURFACE_STYLE_FILL_AREA(#10411);
#10413=SURFACE_SIDE_STYLE('',(#10412));
#10414=SURFACE_STYLE_USAGE(.BOTH.,#10413);
#10415=PRESENTATION_STYLE_ASSIGNMENT((#10414));
ENDSEC;
END-ISO-10303-21;
